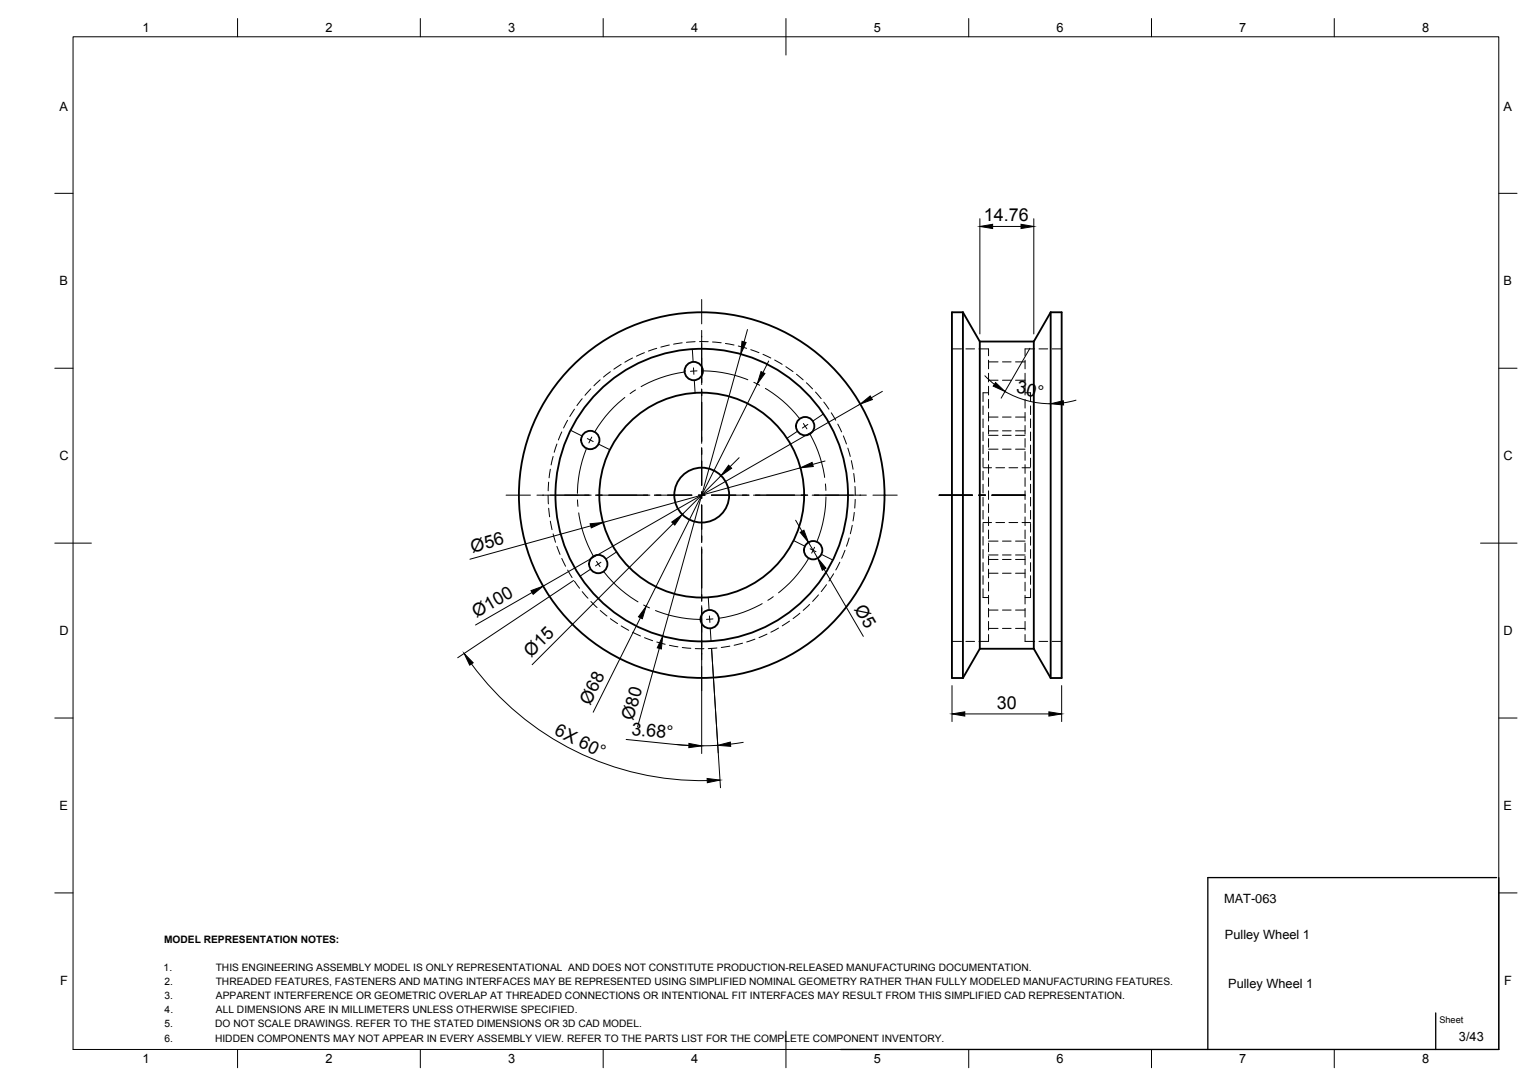
ISO-10303-21;
HEADER;
/* Generated by software containing ST-Developer
 * from STEP Tools, Inc. (www.steptools.com) 
 */

FILE_DESCRIPTION(
/* description */ (''),
/* implementation_level */ '2;1');

FILE_NAME(
/* name */ 'Pulley Wheel 1.step',
/* time_stamp */ '2026-10-24T09:43:01-07:00',
/* author */ (''),
/* organization */ (''),
/* preprocessor_version */ 'ST-DEVELOPER v20.2',
/* originating_system */ 'Autodesk Translation Framework v15.15.0.0',
/* authorisation */ '');

FILE_SCHEMA (('AUTOMOTIVE_DESIGN { 1 0 10303 214 3 1 1 }'));
ENDSEC;

DATA;
#10=MECHANICAL_DESIGN_GEOMETRIC_PRESENTATION_REPRESENTATION('',(#273),#11112);
#207=SHAPE_REPRESENTATION_RELATIONSHIP('SRR','None',#11230,#240);
#240=ADVANCED_BREP_SHAPE_REPRESENTATION('',(#306),#11075);
#273=STYLED_ITEM('',(#11424),#306);
#306=MANIFOLD_SOLID_BREP('Pulley Wheel 1',#6010);
#339=FACE_BOUND('',#1044,.T.);
#340=FACE_BOUND('',#1046,.T.);
#341=FACE_BOUND('',#1050,.T.);
#342=FACE_BOUND('',#1051,.T.);
#343=FACE_BOUND('',#1052,.T.);
#344=FACE_BOUND('',#1053,.T.);
#345=FACE_BOUND('',#1054,.T.);
#346=FACE_BOUND('',#1055,.T.);
#347=FACE_BOUND('',#1056,.T.);
#348=FACE_BOUND('',#1058,.T.);
#349=FACE_BOUND('',#1059,.T.);
#350=FACE_BOUND('',#1060,.T.);
#351=FACE_BOUND('',#1061,.T.);
#352=FACE_BOUND('',#1062,.T.);
#353=FACE_BOUND('',#1063,.T.);
#354=FACE_BOUND('',#1064,.T.);
#355=FACE_BOUND('',#1074,.T.);
#356=FACE_BOUND('',#1076,.T.);
#496=PLANE('',#6425);
#497=PLANE('',#6427);
#498=PLANE('',#6433);
#499=PLANE('',#6441);
#500=PLANE('',#6459);
#501=PLANE('',#6460);
#665=CONICAL_SURFACE('',#6416,1.,1.04719756558882);
#666=CONICAL_SURFACE('',#6418,1.,1.04719756558882);
#673=FACE_OUTER_BOUND('',#1037,.T.);
#674=FACE_OUTER_BOUND('',#1038,.T.);
#675=FACE_OUTER_BOUND('',#1039,.T.);
#676=FACE_OUTER_BOUND('',#1040,.T.);
#677=FACE_OUTER_BOUND('',#1041,.T.);
#678=FACE_OUTER_BOUND('',#1042,.T.);
#679=FACE_OUTER_BOUND('',#1043,.T.);
#680=FACE_OUTER_BOUND('',#1045,.T.);
#681=FACE_OUTER_BOUND('',#1047,.T.);
#682=FACE_OUTER_BOUND('',#1048,.T.);
#683=FACE_OUTER_BOUND('',#1049,.T.);
#684=FACE_OUTER_BOUND('',#1057,.T.);
#685=FACE_OUTER_BOUND('',#1065,.T.);
#686=FACE_OUTER_BOUND('',#1066,.T.);
#687=FACE_OUTER_BOUND('',#1067,.T.);
#688=FACE_OUTER_BOUND('',#1068,.T.);
#689=FACE_OUTER_BOUND('',#1069,.T.);
#690=FACE_OUTER_BOUND('',#1070,.T.);
#691=FACE_OUTER_BOUND('',#1071,.T.);
#692=FACE_OUTER_BOUND('',#1072,.T.);
#693=FACE_OUTER_BOUND('',#1073,.T.);
#694=FACE_OUTER_BOUND('',#1075,.T.);
#1037=EDGE_LOOP('',(#3953,#3954,#3955,#3956));
#1038=EDGE_LOOP('',(#3957,#3958,#3959,#3960,#3961));
#1039=EDGE_LOOP('',(#3962,#3963,#3964,#3965,#3966));
#1040=EDGE_LOOP('',(#3967,#3968,#3969,#3970,#3971));
#1041=EDGE_LOOP('',(#3972,#3973,#3974,#3975));
#1042=EDGE_LOOP('',(#3976,#3977,#3978,#3979,#3980));
#1043=EDGE_LOOP('',(#3981));
#1044=EDGE_LOOP('',(#3982));
#1045=EDGE_LOOP('',(#3983));
#1046=EDGE_LOOP('',(#3984));
#1047=EDGE_LOOP('',(#3985,#3986,#3987,#3988));
#1048=EDGE_LOOP('',(#3989,#3990,#3991,#3992));
#1049=EDGE_LOOP('',(#3993));
#1050=EDGE_LOOP('',(#3994));
#1051=EDGE_LOOP('',(#3995));
#1052=EDGE_LOOP('',(#3996));
#1053=EDGE_LOOP('',(#3997));
#1054=EDGE_LOOP('',(#3998));
#1055=EDGE_LOOP('',(#3999));
#1056=EDGE_LOOP('',(#4000));
#1057=EDGE_LOOP('',(#4001));
#1058=EDGE_LOOP('',(#4002));
#1059=EDGE_LOOP('',(#4003));
#1060=EDGE_LOOP('',(#4004));
#1061=EDGE_LOOP('',(#4005));
#1062=EDGE_LOOP('',(#4006));
#1063=EDGE_LOOP('',(#4007));
#1064=EDGE_LOOP('',(#4008));
#1065=EDGE_LOOP('',(#4009,#4010,#4011,#4012));
#1066=EDGE_LOOP('',(#4013,#4014,#4015,#4016));
#1067=EDGE_LOOP('',(#4017,#4018,#4019,#4020));
#1068=EDGE_LOOP('',(#4021,#4022,#4023,#4024));
#1069=EDGE_LOOP('',(#4025,#4026,#4027,#4028));
#1070=EDGE_LOOP('',(#4029,#4030,#4031,#4032));
#1071=EDGE_LOOP('',(#4033,#4034,#4035,#4036));
#1072=EDGE_LOOP('',(#4037,#4038,#4039,#4040));
#1073=EDGE_LOOP('',(#4041));
#1074=EDGE_LOOP('',(#4042));
#1075=EDGE_LOOP('',(#4043));
#1076=EDGE_LOOP('',(#4044));
#1558=LINE('',#9331,#1917);
#1559=LINE('',#9337,#1918);
#1560=LINE('',#9344,#1919);
#1561=LINE('',#9349,#1920);
#1562=LINE('',#9354,#1921);
#1563=LINE('',#9357,#1922);
#1564=LINE('',#9368,#1923);
#1565=LINE('',#9371,#1924);
#1566=LINE('',#9406,#1925);
#1567=LINE('',#9408,#1926);
#1568=LINE('',#9410,#1927);
#1569=LINE('',#9412,#1928);
#1570=LINE('',#9414,#1929);
#1571=LINE('',#9416,#1930);
#1572=LINE('',#9418,#1931);
#1573=LINE('',#9421,#1932);
#1917=VECTOR('',#7268,0.00749999975240882);
#1918=VECTOR('',#7275,0.042);
#1919=VECTOR('',#7284,1.);
#1920=VECTOR('',#7289,1.);
#1921=VECTOR('',#7296,0.05);
#1922=VECTOR('',#7299,0.05);
#1923=VECTOR('',#7314,0.04);
#1924=VECTOR('',#7317,0.04);
#1925=VECTOR('',#7356,0.028);
#1926=VECTOR('',#7359,0.0025);
#1927=VECTOR('',#7362,0.0025);
#1928=VECTOR('',#7365,0.0025);
#1929=VECTOR('',#7368,0.0025);
#1930=VECTOR('',#7371,0.0025);
#1931=VECTOR('',#7374,0.0025);
#1932=VECTOR('',#7377,0.028);
#2276=CIRCLE('',#6410,0.00749999975240882);
#2277=CIRCLE('',#6411,0.00749999975240882);
#2278=CIRCLE('',#6413,0.042);
#2279=CIRCLE('',#6414,0.042);
#2280=CIRCLE('',#6415,0.042);
#2281=CIRCLE('',#6417,0.05);
#2282=CIRCLE('',#6419,0.05);
#2283=CIRCLE('',#6420,0.05);
#2284=CIRCLE('',#6422,0.05);
#2285=CIRCLE('',#6424,0.05);
#2286=CIRCLE('',#6426,0.04);
#2287=CIRCLE('',#6428,0.04);
#2288=CIRCLE('',#6430,0.04);
#2289=CIRCLE('',#6432,0.04);
#2290=CIRCLE('',#6434,0.0025);
#2291=CIRCLE('',#6435,0.0025);
#2292=CIRCLE('',#6436,0.0025);
#2293=CIRCLE('',#6437,0.0025);
#2294=CIRCLE('',#6438,0.0025);
#2295=CIRCLE('',#6439,0.0025);
#2296=CIRCLE('',#6440,0.028);
#2297=CIRCLE('',#6442,0.0025);
#2298=CIRCLE('',#6443,0.0025);
#2299=CIRCLE('',#6444,0.0025);
#2300=CIRCLE('',#6445,0.0025);
#2301=CIRCLE('',#6446,0.0025);
#2302=CIRCLE('',#6447,0.0025);
#2303=CIRCLE('',#6448,0.028);
#2304=CIRCLE('',#6450,0.028);
#2305=CIRCLE('',#6458,0.028);
#2682=VERTEX_POINT('',#9328);
#2683=VERTEX_POINT('',#9330);
#2684=VERTEX_POINT('',#9334);
#2685=VERTEX_POINT('',#9336);
#2686=VERTEX_POINT('',#9338);
#2687=VERTEX_POINT('',#9342);
#2688=VERTEX_POINT('',#9346);
#2689=VERTEX_POINT('',#9347);
#2690=VERTEX_POINT('',#9352);
#2691=VERTEX_POINT('',#9356);
#2692=VERTEX_POINT('',#9360);
#2693=VERTEX_POINT('',#9363);
#2694=VERTEX_POINT('',#9366);
#2695=VERTEX_POINT('',#9370);
#2696=VERTEX_POINT('',#9374);
#2697=VERTEX_POINT('',#9376);
#2698=VERTEX_POINT('',#9378);
#2699=VERTEX_POINT('',#9380);
#2700=VERTEX_POINT('',#9382);
#2701=VERTEX_POINT('',#9384);
#2702=VERTEX_POINT('',#9386);
#2703=VERTEX_POINT('',#9389);
#2704=VERTEX_POINT('',#9391);
#2705=VERTEX_POINT('',#9393);
#2706=VERTEX_POINT('',#9395);
#2707=VERTEX_POINT('',#9397);
#2708=VERTEX_POINT('',#9399);
#2709=VERTEX_POINT('',#9401);
#2710=VERTEX_POINT('',#9404);
#2711=VERTEX_POINT('',#9420);
#3180=EDGE_CURVE('',#2682,#2682,#2276,.T.);
#3181=EDGE_CURVE('',#2682,#2683,#1558,.T.);
#3182=EDGE_CURVE('',#2683,#2683,#2277,.T.);
#3183=EDGE_CURVE('',#2684,#2684,#2278,.F.);
#3184=EDGE_CURVE('',#2684,#2685,#1559,.T.);
#3185=EDGE_CURVE('',#2685,#2686,#2279,.F.);
#3186=EDGE_CURVE('',#2686,#2685,#2280,.F.);
#3187=EDGE_CURVE('',#2687,#2687,#2281,.F.);
#3188=EDGE_CURVE('',#2687,#2686,#1560,.T.);
#3189=EDGE_CURVE('',#2688,#2689,#2282,.F.);
#3190=EDGE_CURVE('',#2689,#2684,#1561,.T.);
#3191=EDGE_CURVE('',#2689,#2688,#2283,.F.);
#3192=EDGE_CURVE('',#2690,#2690,#2284,.F.);
#3193=EDGE_CURVE('',#2690,#2687,#1562,.T.);
#3194=EDGE_CURVE('',#2688,#2691,#1563,.T.);
#3195=EDGE_CURVE('',#2691,#2691,#2285,.T.);
#3196=EDGE_CURVE('',#2692,#2692,#2286,.T.);
#3197=EDGE_CURVE('',#2693,#2693,#2287,.T.);
#3198=EDGE_CURVE('',#2694,#2694,#2288,.T.);
#3199=EDGE_CURVE('',#2694,#2692,#1564,.T.);
#3200=EDGE_CURVE('',#2693,#2695,#1565,.T.);
#3201=EDGE_CURVE('',#2695,#2695,#2289,.F.);
#3202=EDGE_CURVE('',#2696,#2696,#2290,.F.);
#3203=EDGE_CURVE('',#2697,#2697,#2291,.F.);
#3204=EDGE_CURVE('',#2698,#2698,#2292,.F.);
#3205=EDGE_CURVE('',#2699,#2699,#2293,.F.);
#3206=EDGE_CURVE('',#2700,#2700,#2294,.F.);
#3207=EDGE_CURVE('',#2701,#2701,#2295,.F.);
#3208=EDGE_CURVE('',#2702,#2702,#2296,.T.);
#3209=EDGE_CURVE('',#2703,#2703,#2297,.F.);
#3210=EDGE_CURVE('',#2704,#2704,#2298,.F.);
#3211=EDGE_CURVE('',#2705,#2705,#2299,.F.);
#3212=EDGE_CURVE('',#2706,#2706,#2300,.F.);
#3213=EDGE_CURVE('',#2707,#2707,#2301,.F.);
#3214=EDGE_CURVE('',#2708,#2708,#2302,.F.);
#3215=EDGE_CURVE('',#2709,#2709,#2303,.T.);
#3216=EDGE_CURVE('',#2710,#2710,#2304,.F.);
#3217=EDGE_CURVE('',#2710,#2702,#1566,.T.);
#3218=EDGE_CURVE('',#2701,#2708,#1567,.T.);
#3219=EDGE_CURVE('',#2700,#2707,#1568,.T.);
#3220=EDGE_CURVE('',#2699,#2706,#1569,.T.);
#3221=EDGE_CURVE('',#2698,#2705,#1570,.T.);
#3222=EDGE_CURVE('',#2697,#2704,#1571,.T.);
#3223=EDGE_CURVE('',#2696,#2703,#1572,.T.);
#3224=EDGE_CURVE('',#2709,#2711,#1573,.T.);
#3225=EDGE_CURVE('',#2711,#2711,#2305,.T.);
#3953=ORIENTED_EDGE('',*,*,#3180,.T.);
#3954=ORIENTED_EDGE('',*,*,#3181,.T.);
#3955=ORIENTED_EDGE('',*,*,#3182,.F.);
#3956=ORIENTED_EDGE('',*,*,#3181,.F.);
#3957=ORIENTED_EDGE('',*,*,#3183,.T.);
#3958=ORIENTED_EDGE('',*,*,#3184,.T.);
#3959=ORIENTED_EDGE('',*,*,#3185,.T.);
#3960=ORIENTED_EDGE('',*,*,#3186,.T.);
#3961=ORIENTED_EDGE('',*,*,#3184,.F.);
#3962=ORIENTED_EDGE('',*,*,#3187,.T.);
#3963=ORIENTED_EDGE('',*,*,#3188,.T.);
#3964=ORIENTED_EDGE('',*,*,#3185,.F.);
#3965=ORIENTED_EDGE('',*,*,#3186,.F.);
#3966=ORIENTED_EDGE('',*,*,#3188,.F.);
#3967=ORIENTED_EDGE('',*,*,#3189,.T.);
#3968=ORIENTED_EDGE('',*,*,#3190,.T.);
#3969=ORIENTED_EDGE('',*,*,#3183,.F.);
#3970=ORIENTED_EDGE('',*,*,#3190,.F.);
#3971=ORIENTED_EDGE('',*,*,#3191,.T.);
#3972=ORIENTED_EDGE('',*,*,#3192,.T.);
#3973=ORIENTED_EDGE('',*,*,#3193,.T.);
#3974=ORIENTED_EDGE('',*,*,#3187,.F.);
#3975=ORIENTED_EDGE('',*,*,#3193,.F.);
#3976=ORIENTED_EDGE('',*,*,#3189,.F.);
#3977=ORIENTED_EDGE('',*,*,#3194,.T.);
#3978=ORIENTED_EDGE('',*,*,#3195,.T.);
#3979=ORIENTED_EDGE('',*,*,#3194,.F.);
#3980=ORIENTED_EDGE('',*,*,#3191,.F.);
#3981=ORIENTED_EDGE('',*,*,#3192,.F.);
#3982=ORIENTED_EDGE('',*,*,#3196,.F.);
#3983=ORIENTED_EDGE('',*,*,#3195,.F.);
#3984=ORIENTED_EDGE('',*,*,#3197,.T.);
#3985=ORIENTED_EDGE('',*,*,#3198,.F.);
#3986=ORIENTED_EDGE('',*,*,#3199,.T.);
#3987=ORIENTED_EDGE('',*,*,#3196,.T.);
#3988=ORIENTED_EDGE('',*,*,#3199,.F.);
#3989=ORIENTED_EDGE('',*,*,#3197,.F.);
#3990=ORIENTED_EDGE('',*,*,#3200,.T.);
#3991=ORIENTED_EDGE('',*,*,#3201,.F.);
#3992=ORIENTED_EDGE('',*,*,#3200,.F.);
#3993=ORIENTED_EDGE('',*,*,#3198,.T.);
#3994=ORIENTED_EDGE('',*,*,#3202,.F.);
#3995=ORIENTED_EDGE('',*,*,#3203,.F.);
#3996=ORIENTED_EDGE('',*,*,#3204,.F.);
#3997=ORIENTED_EDGE('',*,*,#3205,.F.);
#3998=ORIENTED_EDGE('',*,*,#3206,.F.);
#3999=ORIENTED_EDGE('',*,*,#3207,.F.);
#4000=ORIENTED_EDGE('',*,*,#3208,.F.);
#4001=ORIENTED_EDGE('',*,*,#3201,.T.);
#4002=ORIENTED_EDGE('',*,*,#3209,.T.);
#4003=ORIENTED_EDGE('',*,*,#3210,.T.);
#4004=ORIENTED_EDGE('',*,*,#3211,.T.);
#4005=ORIENTED_EDGE('',*,*,#3212,.T.);
#4006=ORIENTED_EDGE('',*,*,#3213,.T.);
#4007=ORIENTED_EDGE('',*,*,#3214,.T.);
#4008=ORIENTED_EDGE('',*,*,#3215,.T.);
#4009=ORIENTED_EDGE('',*,*,#3216,.T.);
#4010=ORIENTED_EDGE('',*,*,#3217,.T.);
#4011=ORIENTED_EDGE('',*,*,#3208,.T.);
#4012=ORIENTED_EDGE('',*,*,#3217,.F.);
#4013=ORIENTED_EDGE('',*,*,#3207,.T.);
#4014=ORIENTED_EDGE('',*,*,#3218,.T.);
#4015=ORIENTED_EDGE('',*,*,#3214,.F.);
#4016=ORIENTED_EDGE('',*,*,#3218,.F.);
#4017=ORIENTED_EDGE('',*,*,#3206,.T.);
#4018=ORIENTED_EDGE('',*,*,#3219,.T.);
#4019=ORIENTED_EDGE('',*,*,#3213,.F.);
#4020=ORIENTED_EDGE('',*,*,#3219,.F.);
#4021=ORIENTED_EDGE('',*,*,#3205,.T.);
#4022=ORIENTED_EDGE('',*,*,#3220,.T.);
#4023=ORIENTED_EDGE('',*,*,#3212,.F.);
#4024=ORIENTED_EDGE('',*,*,#3220,.F.);
#4025=ORIENTED_EDGE('',*,*,#3204,.T.);
#4026=ORIENTED_EDGE('',*,*,#3221,.T.);
#4027=ORIENTED_EDGE('',*,*,#3211,.F.);
#4028=ORIENTED_EDGE('',*,*,#3221,.F.);
#4029=ORIENTED_EDGE('',*,*,#3203,.T.);
#4030=ORIENTED_EDGE('',*,*,#3222,.T.);
#4031=ORIENTED_EDGE('',*,*,#3210,.F.);
#4032=ORIENTED_EDGE('',*,*,#3222,.F.);
#4033=ORIENTED_EDGE('',*,*,#3202,.T.);
#4034=ORIENTED_EDGE('',*,*,#3223,.T.);
#4035=ORIENTED_EDGE('',*,*,#3209,.F.);
#4036=ORIENTED_EDGE('',*,*,#3223,.F.);
#4037=ORIENTED_EDGE('',*,*,#3215,.F.);
#4038=ORIENTED_EDGE('',*,*,#3224,.T.);
#4039=ORIENTED_EDGE('',*,*,#3225,.T.);
#4040=ORIENTED_EDGE('',*,*,#3224,.F.);
#4041=ORIENTED_EDGE('',*,*,#3216,.F.);
#4042=ORIENTED_EDGE('',*,*,#3182,.T.);
#4043=ORIENTED_EDGE('',*,*,#3225,.F.);
#4044=ORIENTED_EDGE('',*,*,#3180,.F.);
#5499=CYLINDRICAL_SURFACE('',#6409,0.00749999975240882);
#5500=CYLINDRICAL_SURFACE('',#6412,0.042);
#5501=CYLINDRICAL_SURFACE('',#6421,0.05);
#5502=CYLINDRICAL_SURFACE('',#6423,0.05);
#5503=CYLINDRICAL_SURFACE('',#6429,0.04);
#5504=CYLINDRICAL_SURFACE('',#6431,0.04);
#5505=CYLINDRICAL_SURFACE('',#6449,0.028);
#5506=CYLINDRICAL_SURFACE('',#6451,0.0025);
#5507=CYLINDRICAL_SURFACE('',#6452,0.0025);
#5508=CYLINDRICAL_SURFACE('',#6453,0.0025);
#5509=CYLINDRICAL_SURFACE('',#6454,0.0025);
#5510=CYLINDRICAL_SURFACE('',#6455,0.0025);
#5511=CYLINDRICAL_SURFACE('',#6456,0.0025);
#5512=CYLINDRICAL_SURFACE('',#6457,0.028);
#5646=ADVANCED_FACE('',(#673),#5499,.F.);
#5647=ADVANCED_FACE('',(#674),#5500,.T.);
#5648=ADVANCED_FACE('',(#675),#665,.T.);
#5649=ADVANCED_FACE('',(#676),#666,.T.);
#5650=ADVANCED_FACE('',(#677),#5501,.T.);
#5651=ADVANCED_FACE('',(#678),#5502,.T.);
#5652=ADVANCED_FACE('',(#679,#339),#496,.F.);
#5653=ADVANCED_FACE('',(#680,#340),#497,.T.);
#5654=ADVANCED_FACE('',(#681),#5503,.F.);
#5655=ADVANCED_FACE('',(#682),#5504,.F.);
#5656=ADVANCED_FACE('',(#683,#341,#342,#343,#344,#345,#346,#347),#498,.F.);
#5657=ADVANCED_FACE('',(#684,#348,#349,#350,#351,#352,#353,#354),#499,.T.);
#5658=ADVANCED_FACE('',(#685),#5505,.T.);
#5659=ADVANCED_FACE('',(#686),#5506,.F.);
#5660=ADVANCED_FACE('',(#687),#5507,.F.);
#5661=ADVANCED_FACE('',(#688),#5508,.F.);
#5662=ADVANCED_FACE('',(#689),#5509,.F.);
#5663=ADVANCED_FACE('',(#690),#5510,.F.);
#5664=ADVANCED_FACE('',(#691),#5511,.F.);
#5665=ADVANCED_FACE('',(#692),#5512,.T.);
#5666=ADVANCED_FACE('',(#693,#355),#500,.F.);
#5667=ADVANCED_FACE('',(#694,#356),#501,.T.);
#6010=CLOSED_SHELL('',(#5646,#5647,#5648,#5649,#5650,#5651,#5652,#5653,
#5654,#5655,#5656,#5657,#5658,#5659,#5660,#5661,#5662,#5663,#5664,#5665,
#5666,#5667));
#6408=AXIS2_PLACEMENT_3D('',#9326,#7262,#7263);
#6409=AXIS2_PLACEMENT_3D('',#9327,#7264,#7265);
#6410=AXIS2_PLACEMENT_3D('',#9329,#7266,#7267);
#6411=AXIS2_PLACEMENT_3D('',#9332,#7269,#7270);
#6412=AXIS2_PLACEMENT_3D('',#9333,#7271,#7272);
#6413=AXIS2_PLACEMENT_3D('',#9335,#7273,#7274);
#6414=AXIS2_PLACEMENT_3D('',#9339,#7276,#7277);
#6415=AXIS2_PLACEMENT_3D('',#9340,#7278,#7279);
#6416=AXIS2_PLACEMENT_3D('',#9341,#7280,#7281);
#6417=AXIS2_PLACEMENT_3D('',#9343,#7282,#7283);
#6418=AXIS2_PLACEMENT_3D('',#9345,#7285,#7286);
#6419=AXIS2_PLACEMENT_3D('',#9348,#7287,#7288);
#6420=AXIS2_PLACEMENT_3D('',#9350,#7290,#7291);
#6421=AXIS2_PLACEMENT_3D('',#9351,#7292,#7293);
#6422=AXIS2_PLACEMENT_3D('',#9353,#7294,#7295);
#6423=AXIS2_PLACEMENT_3D('',#9355,#7297,#7298);
#6424=AXIS2_PLACEMENT_3D('',#9358,#7300,#7301);
#6425=AXIS2_PLACEMENT_3D('',#9359,#7302,#7303);
#6426=AXIS2_PLACEMENT_3D('',#9361,#7304,#7305);
#6427=AXIS2_PLACEMENT_3D('',#9362,#7306,#7307);
#6428=AXIS2_PLACEMENT_3D('',#9364,#7308,#7309);
#6429=AXIS2_PLACEMENT_3D('',#9365,#7310,#7311);
#6430=AXIS2_PLACEMENT_3D('',#9367,#7312,#7313);
#6431=AXIS2_PLACEMENT_3D('',#9369,#7315,#7316);
#6432=AXIS2_PLACEMENT_3D('',#9372,#7318,#7319);
#6433=AXIS2_PLACEMENT_3D('',#9373,#7320,#7321);
#6434=AXIS2_PLACEMENT_3D('',#9375,#7322,#7323);
#6435=AXIS2_PLACEMENT_3D('',#9377,#7324,#7325);
#6436=AXIS2_PLACEMENT_3D('',#9379,#7326,#7327);
#6437=AXIS2_PLACEMENT_3D('',#9381,#7328,#7329);
#6438=AXIS2_PLACEMENT_3D('',#9383,#7330,#7331);
#6439=AXIS2_PLACEMENT_3D('',#9385,#7332,#7333);
#6440=AXIS2_PLACEMENT_3D('',#9387,#7334,#7335);
#6441=AXIS2_PLACEMENT_3D('',#9388,#7336,#7337);
#6442=AXIS2_PLACEMENT_3D('',#9390,#7338,#7339);
#6443=AXIS2_PLACEMENT_3D('',#9392,#7340,#7341);
#6444=AXIS2_PLACEMENT_3D('',#9394,#7342,#7343);
#6445=AXIS2_PLACEMENT_3D('',#9396,#7344,#7345);
#6446=AXIS2_PLACEMENT_3D('',#9398,#7346,#7347);
#6447=AXIS2_PLACEMENT_3D('',#9400,#7348,#7349);
#6448=AXIS2_PLACEMENT_3D('',#9402,#7350,#7351);
#6449=AXIS2_PLACEMENT_3D('',#9403,#7352,#7353);
#6450=AXIS2_PLACEMENT_3D('',#9405,#7354,#7355);
#6451=AXIS2_PLACEMENT_3D('',#9407,#7357,#7358);
#6452=AXIS2_PLACEMENT_3D('',#9409,#7360,#7361);
#6453=AXIS2_PLACEMENT_3D('',#9411,#7363,#7364);
#6454=AXIS2_PLACEMENT_3D('',#9413,#7366,#7367);
#6455=AXIS2_PLACEMENT_3D('',#9415,#7369,#7370);
#6456=AXIS2_PLACEMENT_3D('',#9417,#7372,#7373);
#6457=AXIS2_PLACEMENT_3D('',#9419,#7375,#7376);
#6458=AXIS2_PLACEMENT_3D('',#9422,#7378,#7379);
#6459=AXIS2_PLACEMENT_3D('',#9423,#7380,#7381);
#6460=AXIS2_PLACEMENT_3D('',#9424,#7382,#7383);
#7262=DIRECTION('axis',(0.,0.,1.));
#7263=DIRECTION('refdir',(1.,0.,0.));
#7264=DIRECTION('center_axis',(0.,0.,1.));
#7265=DIRECTION('ref_axis',(1.,1.37975427514318E-9,0.));
#7266=DIRECTION('center_axis',(6.39458016332861E-18,1.10411609048463E-17,
1.));
#7267=DIRECTION('ref_axis',(1.,1.37975427514318E-9,0.));
#7268=DIRECTION('',(0.,0.,-1.));
#7269=DIRECTION('center_axis',(0.,0.,1.));
#7270=DIRECTION('ref_axis',(1.,1.37975427514318E-9,0.));
#7271=DIRECTION('center_axis',(4.13029399042097E-17,0.,1.));
#7272=DIRECTION('ref_axis',(1.,0.,-4.13029399042097E-17));
#7273=DIRECTION('center_axis',(-3.04809470411818E-27,2.64338815530979E-17,
1.));
#7274=DIRECTION('ref_axis',(1.,-4.29586510583046E-10,0.));
#7275=DIRECTION('',(-4.13029399042097E-17,0.,-1.));
#7276=DIRECTION('center_axis',(-5.28677630773884E-17,-1.0843360466812E-26,
-1.));
#7277=DIRECTION('ref_axis',(1.,2.50000086925735E-10,-5.28677630773884E-17));
#7278=DIRECTION('center_axis',(-5.28677630773884E-17,-1.0843360466812E-26,
-1.));
#7279=DIRECTION('ref_axis',(1.,2.50000086925735E-10,-5.28677630773884E-17));
#7280=DIRECTION('center_axis',(-1.70140119462979E-16,0.,-1.));
#7281=DIRECTION('ref_axis',(-1.,0.,1.70140119462979E-16));
#7282=DIRECTION('center_axis',(-9.76996261870523E-16,-9.7699626151362E-16,
-1.));
#7283=DIRECTION('ref_axis',(1.,-1.60206417040051E-10,-9.76996261670138E-16));
#7284=DIRECTION('',(-0.86602541098055,1.0605752475376E-16,0.49999998753597));
#7285=DIRECTION('center_axis',(1.70140119462979E-16,0.,1.));
#7286=DIRECTION('ref_axis',(1.,0.,-1.70140119462979E-16));
#7287=DIRECTION('center_axis',(0.,0.,1.));
#7288=DIRECTION('ref_axis',(-1.,-1.60206710118277E-10,0.));
#7289=DIRECTION('',(0.86602541098055,1.0605752475376E-16,-0.49999998753597));
#7290=DIRECTION('center_axis',(0.,0.,1.));
#7291=DIRECTION('ref_axis',(-1.,-1.60206710118277E-10,0.));
#7292=DIRECTION('center_axis',(0.,0.,-1.));
#7293=DIRECTION('ref_axis',(-1.,0.,0.));
#7294=DIRECTION('center_axis',(0.,0.,-1.));
#7295=DIRECTION('ref_axis',(-1.,0.,0.));
#7296=DIRECTION('',(0.,0.,1.));
#7297=DIRECTION('center_axis',(0.,0.,-1.));
#7298=DIRECTION('ref_axis',(-1.,0.,0.));
#7299=DIRECTION('',(0.,0.,1.));
#7300=DIRECTION('center_axis',(0.,0.,-1.));
#7301=DIRECTION('ref_axis',(-1.,0.,0.));
#7302=DIRECTION('center_axis',(2.84990285479818E-18,3.64291930135101E-18,
1.));
#7303=DIRECTION('ref_axis',(0.,-1.,3.64291930135101E-18));
#7304=DIRECTION('center_axis',(-2.16840434497101E-17,0.,-1.));
#7305=DIRECTION('ref_axis',(-1.,0.,2.16840434497101E-17));
#7306=DIRECTION('center_axis',(-2.84990285479818E-18,-3.64291930135101E-18,
1.));
#7307=DIRECTION('ref_axis',(0.,-1.,-3.64291930135101E-18));
#7308=DIRECTION('center_axis',(0.,0.,-1.));
#7309=DIRECTION('ref_axis',(-1.,0.,0.));
#7310=DIRECTION('center_axis',(-2.16840434497101E-17,0.,-1.));
#7311=DIRECTION('ref_axis',(-1.,0.,2.16840434497101E-17));
#7312=DIRECTION('center_axis',(-2.16840434497101E-17,0.,-1.));
#7313=DIRECTION('ref_axis',(-1.,0.,2.16840434497101E-17));
#7314=DIRECTION('',(-2.16840434497101E-17,0.,-1.));
#7315=DIRECTION('center_axis',(0.,0.,-1.));
#7316=DIRECTION('ref_axis',(-1.,0.,0.));
#7317=DIRECTION('',(0.,0.,-1.));
#7318=DIRECTION('center_axis',(0.,0.,-1.));
#7319=DIRECTION('ref_axis',(-1.,0.,0.));
#7320=DIRECTION('center_axis',(-6.27288400105048E-18,-2.92734586715581E-18,
1.));
#7321=DIRECTION('ref_axis',(1.,-1.25733582200228E-51,6.27288400105048E-18));
#7322=DIRECTION('center_axis',(-3.46944695195361E-16,0.,1.));
#7323=DIRECTION('ref_axis',(1.,0.,3.46944695195361E-16));
#7324=DIRECTION('center_axis',(-3.46944695195361E-16,0.,1.));
#7325=DIRECTION('ref_axis',(1.,0.,3.46944695195361E-16));
#7326=DIRECTION('center_axis',(-3.46944695195362E-16,0.,1.));
#7327=DIRECTION('ref_axis',(1.,0.,3.46944695195362E-16));
#7328=DIRECTION('center_axis',(-3.46944695195361E-16,0.,1.));
#7329=DIRECTION('ref_axis',(1.,0.,3.46944695195361E-16));
#7330=DIRECTION('center_axis',(-3.46944695195361E-16,0.,1.));
#7331=DIRECTION('ref_axis',(1.,0.,3.46944695195361E-16));
#7332=DIRECTION('center_axis',(-3.46944695195362E-16,0.,1.));
#7333=DIRECTION('ref_axis',(1.,0.,3.46944695195362E-16));
#7334=DIRECTION('center_axis',(0.,0.,-1.));
#7335=DIRECTION('ref_axis',(-1.,0.,0.));
#7336=DIRECTION('center_axis',(6.27288400105048E-18,2.92734586715581E-18,
1.));
#7337=DIRECTION('ref_axis',(1.,-1.25733582200228E-51,-6.27288400105048E-18));
#7338=DIRECTION('center_axis',(-3.46944695195361E-16,0.,1.));
#7339=DIRECTION('ref_axis',(1.,0.,3.46944695195361E-16));
#7340=DIRECTION('center_axis',(-3.46944695195361E-16,0.,1.));
#7341=DIRECTION('ref_axis',(1.,0.,3.46944695195361E-16));
#7342=DIRECTION('center_axis',(-3.46944695195362E-16,0.,1.));
#7343=DIRECTION('ref_axis',(1.,0.,3.46944695195362E-16));
#7344=DIRECTION('center_axis',(-3.46944695195361E-16,0.,1.));
#7345=DIRECTION('ref_axis',(1.,0.,3.46944695195361E-16));
#7346=DIRECTION('center_axis',(-3.46944695195361E-16,0.,1.));
#7347=DIRECTION('ref_axis',(1.,0.,3.46944695195361E-16));
#7348=DIRECTION('center_axis',(-3.46944695195362E-16,0.,1.));
#7349=DIRECTION('ref_axis',(1.,0.,3.46944695195362E-16));
#7350=DIRECTION('center_axis',(0.,0.,-1.));
#7351=DIRECTION('ref_axis',(-1.,0.,0.));
#7352=DIRECTION('center_axis',(0.,0.,-1.));
#7353=DIRECTION('ref_axis',(-1.,0.,0.));
#7354=DIRECTION('center_axis',(0.,0.,-1.));
#7355=DIRECTION('ref_axis',(-1.,0.,0.));
#7356=DIRECTION('',(0.,0.,1.));
#7357=DIRECTION('center_axis',(-3.46944695195362E-16,0.,1.));
#7358=DIRECTION('ref_axis',(1.,0.,3.46944695195362E-16));
#7359=DIRECTION('',(-3.46944695195362E-16,0.,1.));
#7360=DIRECTION('center_axis',(-3.46944695195361E-16,0.,1.));
#7361=DIRECTION('ref_axis',(1.,0.,3.46944695195361E-16));
#7362=DIRECTION('',(-3.46944695195361E-16,0.,1.));
#7363=DIRECTION('center_axis',(-3.46944695195361E-16,0.,1.));
#7364=DIRECTION('ref_axis',(1.,0.,3.46944695195361E-16));
#7365=DIRECTION('',(-3.46944695195361E-16,0.,1.));
#7366=DIRECTION('center_axis',(-3.46944695195362E-16,0.,1.));
#7367=DIRECTION('ref_axis',(1.,0.,3.46944695195362E-16));
#7368=DIRECTION('',(-3.46944695195362E-16,0.,1.));
#7369=DIRECTION('center_axis',(-3.46944695195361E-16,0.,1.));
#7370=DIRECTION('ref_axis',(1.,0.,3.46944695195361E-16));
#7371=DIRECTION('',(-3.46944695195361E-16,0.,1.));
#7372=DIRECTION('center_axis',(-3.46944695195361E-16,0.,1.));
#7373=DIRECTION('ref_axis',(1.,0.,3.46944695195361E-16));
#7374=DIRECTION('',(-3.46944695195361E-16,0.,1.));
#7375=DIRECTION('center_axis',(0.,0.,-1.));
#7376=DIRECTION('ref_axis',(-1.,0.,0.));
#7377=DIRECTION('',(0.,0.,1.));
#7378=DIRECTION('center_axis',(0.,0.,-1.));
#7379=DIRECTION('ref_axis',(-1.,0.,0.));
#7380=DIRECTION('center_axis',(-6.39458016332861E-18,-1.10411609048463E-17,
1.));
#7381=DIRECTION('ref_axis',(0.,-1.,-1.10411609048463E-17));
#7382=DIRECTION('center_axis',(6.39458016332861E-18,1.10411609048463E-17,
1.));
#7383=DIRECTION('ref_axis',(0.,-1.,1.10411609048463E-17));
#9326=CARTESIAN_POINT('',(0.,0.,0.));
#9327=CARTESIAN_POINT('Origin',(5.92883964145585E-11,1.19863443615031E-10,
-0.0065));
#9328=CARTESIAN_POINT('',(-0.00749999969312043,1.09515285974588E-10,0.0065));
#9329=CARTESIAN_POINT('Origin',(5.92883964145585E-11,1.19863443615031E-10,
0.0065));
#9330=CARTESIAN_POINT('',(-0.00749999969312043,1.09515287811566E-10,-0.0065));
#9331=CARTESIAN_POINT('',(-0.00749999969312043,1.09515285974588E-10,-0.0065));
#9332=CARTESIAN_POINT('Origin',(5.92883964145585E-11,1.19863443615031E-10,
-0.0065));
#9333=CARTESIAN_POINT('Origin',(-5.74005956283549E-52,0.,0.015));
#9334=CARTESIAN_POINT('',(-0.042,-1.9853686361416E-11,0.007381198));
#9335=CARTESIAN_POINT('Origin',(-2.66453525910038E-17,5.09119415777057E-18,
0.007381198));
#9336=CARTESIAN_POINT('',(-0.042,-1.54820701770975E-11,-0.007381198));
#9337=CARTESIAN_POINT('',(-0.042,-5.14351655641888E-18,0.015));
#9338=CARTESIAN_POINT('',(0.0419999999999985,-5.1435165564187E-18,-0.00738119800000199));
#9339=CARTESIAN_POINT('Origin',(-8.88178419700125E-18,-5.73557577313579E-18,
-0.007381198));
#9340=CARTESIAN_POINT('Origin',(-8.88178419700125E-18,-5.73557577313579E-18,
-0.007381198));
#9341=CARTESIAN_POINT('Origin',(-2.64244881468667E-16,0.,-0.560482737499999));
#9342=CARTESIAN_POINT('',(0.0499999999999997,-6.12323399573673E-18,-0.0120000000000027));
#9343=CARTESIAN_POINT('Origin',(8.88178419700125E-18,1.23918456012259E-18,
-0.012000000000002));
#9344=CARTESIAN_POINT('',(1.,-1.22464679914735E-16,-0.5604827375));
#9345=CARTESIAN_POINT('Origin',(2.63459037944631E-16,0.,0.560482737500119));
#9346=CARTESIAN_POINT('',(0.05,-2.05102985990085E-11,0.0120000000000921));
#9347=CARTESIAN_POINT('',(-0.0499999999999868,-6.12323399573515E-18,0.0120000000001151));
#9348=CARTESIAN_POINT('Origin',(1.77635683940025E-17,-6.31136467490802E-18,
0.0120000000000921));
#9349=CARTESIAN_POINT('',(-1.,-1.22464679914735E-16,0.560482737500119));
#9350=CARTESIAN_POINT('Origin',(1.77635683940025E-17,-6.31136467490802E-18,
0.0120000000000921));
#9351=CARTESIAN_POINT('Origin',(0.,0.,0.015));
#9352=CARTESIAN_POINT('',(0.05,-6.12323399573677E-18,-0.015));
#9353=CARTESIAN_POINT('Origin',(0.,0.,-0.015));
#9354=CARTESIAN_POINT('',(0.05,-6.12323399573677E-18,0.015));
#9355=CARTESIAN_POINT('Origin',(0.,0.,0.015));
#9356=CARTESIAN_POINT('',(0.05,-6.12323399573677E-18,0.015));
#9357=CARTESIAN_POINT('',(0.05,-6.12323399573677E-18,0.015));
#9358=CARTESIAN_POINT('Origin',(0.,0.,0.015));
#9359=CARTESIAN_POINT('Origin',(5.79397640976254E-18,1.73472347597681E-19,
-0.015));
#9360=CARTESIAN_POINT('',(0.04,-4.89858719658941E-18,-0.015));
#9361=CARTESIAN_POINT('Origin',(-6.50521303491303E-19,0.,-0.015));
#9362=CARTESIAN_POINT('Origin',(5.79397640976254E-18,1.73472347597681E-19,
0.015));
#9363=CARTESIAN_POINT('',(0.04,-4.89858719658941E-18,0.015));
#9364=CARTESIAN_POINT('Origin',(0.,0.,0.015));
#9365=CARTESIAN_POINT('Origin',(1.85684700327654E-52,0.,0.015));
#9366=CARTESIAN_POINT('',(0.04,-4.89858719658941E-18,-0.005));
#9367=CARTESIAN_POINT('Origin',(-4.33680868994202E-19,0.,-0.005));
#9368=CARTESIAN_POINT('',(0.04,-4.89858719658941E-18,0.015));
#9369=CARTESIAN_POINT('Origin',(0.,0.,0.015));
#9370=CARTESIAN_POINT('',(0.04,-4.89858719658941E-18,0.005));
#9371=CARTESIAN_POINT('',(0.04,-4.89858719658941E-18,0.015));
#9372=CARTESIAN_POINT('Origin',(0.,0.,0.005));
#9373=CARTESIAN_POINT('Origin',(3.17454396103755E-18,1.73472347597681E-20,
-0.005));
#9374=CARTESIAN_POINT('',(0.026944864,0.017,-0.005));
#9375=CARTESIAN_POINT('Origin',(0.029444864,0.017,-0.005));
#9376=CARTESIAN_POINT('',(0.026944864,-0.017,-0.005));
#9377=CARTESIAN_POINT('Origin',(0.029444864,-0.017,-0.005));
#9378=CARTESIAN_POINT('',(-0.0025,-0.034,-0.005));
#9379=CARTESIAN_POINT('Origin',(-3.46944695195361E-18,-0.034,-0.005));
#9380=CARTESIAN_POINT('',(-0.031944864,-0.017,-0.005));
#9381=CARTESIAN_POINT('Origin',(-0.029444864,-0.017,-0.005));
#9382=CARTESIAN_POINT('',(-0.031944864,0.017,-0.005));
#9383=CARTESIAN_POINT('Origin',(-0.029444864,0.017,-0.005));
#9384=CARTESIAN_POINT('',(-0.0025,0.034,-0.005));
#9385=CARTESIAN_POINT('Origin',(-3.46944695195361E-18,0.034,-0.005));
#9386=CARTESIAN_POINT('',(0.028,-3.42901103761259E-18,-0.005));
#9387=CARTESIAN_POINT('Origin',(0.,0.,-0.005));
#9388=CARTESIAN_POINT('Origin',(3.17454396103755E-18,1.73472347597681E-20,
0.005));
#9389=CARTESIAN_POINT('',(0.026944864,0.017,0.005));
#9390=CARTESIAN_POINT('Origin',(0.029444864,0.017,0.005));
#9391=CARTESIAN_POINT('',(0.026944864,-0.017,0.005));
#9392=CARTESIAN_POINT('Origin',(0.029444864,-0.017,0.005));
#9393=CARTESIAN_POINT('',(-0.00250000000000001,-0.034,0.005));
#9394=CARTESIAN_POINT('Origin',(-6.93889390390723E-18,-0.034,0.005));
#9395=CARTESIAN_POINT('',(-0.031944864,-0.017,0.005));
#9396=CARTESIAN_POINT('Origin',(-0.029444864,-0.017,0.005));
#9397=CARTESIAN_POINT('',(-0.031944864,0.017,0.005));
#9398=CARTESIAN_POINT('Origin',(-0.029444864,0.017,0.005));
#9399=CARTESIAN_POINT('',(-0.00250000000000001,0.034,0.005));
#9400=CARTESIAN_POINT('Origin',(-6.93889390390723E-18,0.034,0.005));
#9401=CARTESIAN_POINT('',(0.028,-3.42901103761259E-18,0.005));
#9402=CARTESIAN_POINT('Origin',(0.,0.,0.005));
#9403=CARTESIAN_POINT('Origin',(0.,0.,0.0065));
#9404=CARTESIAN_POINT('',(0.028,-3.42901103761259E-18,-0.0065));
#9405=CARTESIAN_POINT('Origin',(0.,0.,-0.0065));
#9406=CARTESIAN_POINT('',(0.028,-3.42901103761259E-18,0.0065));
#9407=CARTESIAN_POINT('Origin',(-1.44987137336516E-49,0.034,-0.015));
#9408=CARTESIAN_POINT('',(-0.0025,0.034,-0.015));
#9409=CARTESIAN_POINT('Origin',(-0.029444864,0.017,-0.015));
#9410=CARTESIAN_POINT('',(-0.031944864,0.017,-0.015));
#9411=CARTESIAN_POINT('Origin',(-0.029444864,-0.017,-0.015));
#9412=CARTESIAN_POINT('',(-0.031944864,-0.017,-0.015));
#9413=CARTESIAN_POINT('Origin',(-1.44987137336516E-49,-0.034,-0.015));
#9414=CARTESIAN_POINT('',(-0.0025,-0.034,-0.015));
#9415=CARTESIAN_POINT('Origin',(0.029444864,-0.017,-0.015));
#9416=CARTESIAN_POINT('',(0.026944864,-0.017,-0.015));
#9417=CARTESIAN_POINT('Origin',(0.029444864,0.017,-0.015));
#9418=CARTESIAN_POINT('',(0.026944864,0.017,-0.015));
#9419=CARTESIAN_POINT('Origin',(0.,0.,0.0065));
#9420=CARTESIAN_POINT('',(0.028,-3.42901103761259E-18,0.0065));
#9421=CARTESIAN_POINT('',(0.028,-3.42901103761259E-18,0.0065));
#9422=CARTESIAN_POINT('Origin',(0.,0.,0.0065));
#9423=CARTESIAN_POINT('Origin',(-1.21430643318376E-19,-1.12757025938492E-18,
-0.0065));
#9424=CARTESIAN_POINT('Origin',(-1.21430643318376E-19,-1.12757025938492E-18,
0.0065));
#11036=UNCERTAINTY_MEASURE_WITH_UNIT(LENGTH_MEASURE(1.E-5),#11113,
'DISTANCE_ACCURACY_VALUE',
'Maximum model space distance between geometric entities at asserted c
onnectivities');
#11073=UNCERTAINTY_MEASURE_WITH_UNIT(LENGTH_MEASURE(1.E-5),#11113,
'DISTANCE_ACCURACY_VALUE',
'Maximum model space distance between geometric entities at asserted c
onnectivities');
#11075=(
GEOMETRIC_REPRESENTATION_CONTEXT(3)
GLOBAL_UNCERTAINTY_ASSIGNED_CONTEXT((#11036))
GLOBAL_UNIT_ASSIGNED_CONTEXT((#11113,#11114,#11115))
REPRESENTATION_CONTEXT('','3D')
);
#11112=(
GEOMETRIC_REPRESENTATION_CONTEXT(3)
GLOBAL_UNCERTAINTY_ASSIGNED_CONTEXT((#11073))
GLOBAL_UNIT_ASSIGNED_CONTEXT((#11113,#11114,#11115))
REPRESENTATION_CONTEXT('','3D')
);
#11113=(
LENGTH_UNIT()
NAMED_UNIT(*)
SI_UNIT($,.METRE.)
);
#11114=(
NAMED_UNIT(*)
PLANE_ANGLE_UNIT()
SI_UNIT($,.RADIAN.)
);
#11115=(
NAMED_UNIT(*)
SI_UNIT($,.STERADIAN.)
SOLID_ANGLE_UNIT()
);
#11117=SHAPE_DEFINITION_REPRESENTATION(#11155,#11230);
#11155=PRODUCT_DEFINITION_SHAPE('',$,#11269);
#11230=SHAPE_REPRESENTATION('',(#6408),#11075);
#11267=PRODUCT_DEFINITION_CONTEXT('part definition',#11383,'design');
#11269=PRODUCT_DEFINITION('Pulley Wheel 1','Pulley Wheel 1',#11307,#11267);
#11307=PRODUCT_DEFINITION_FORMATION('',$,#11386);
#11383=APPLICATION_CONTEXT(
'Core Data for Automotive Mechanical Design Process');
#11384=PRODUCT_CONTEXT('part definition',#11383,'mechanical');
#11386=PRODUCT('Pulley Wheel 1','Pulley Wheel 1',
'pulleywheel__ DE    11841',(#11384));
#11424=PRESENTATION_STYLE_ASSIGNMENT((#11428));
#11428=SURFACE_STYLE_USAGE(.BOTH.,#11432);
#11432=SURFACE_SIDE_STYLE('',(#11436));
#11436=SURFACE_STYLE_FILL_AREA(#11440);
#11440=FILL_AREA_STYLE('Opaque(198,193,188)',(#11444));
#11444=FILL_AREA_STYLE_COLOUR('Opaque(198,193,188)',#11448);
#11448=COLOUR_RGB('Opaque(198,193,188)',0.776470588235294,0.756862745098039,
0.737254901960784);
ENDSEC;
END-ISO-10303-21;
